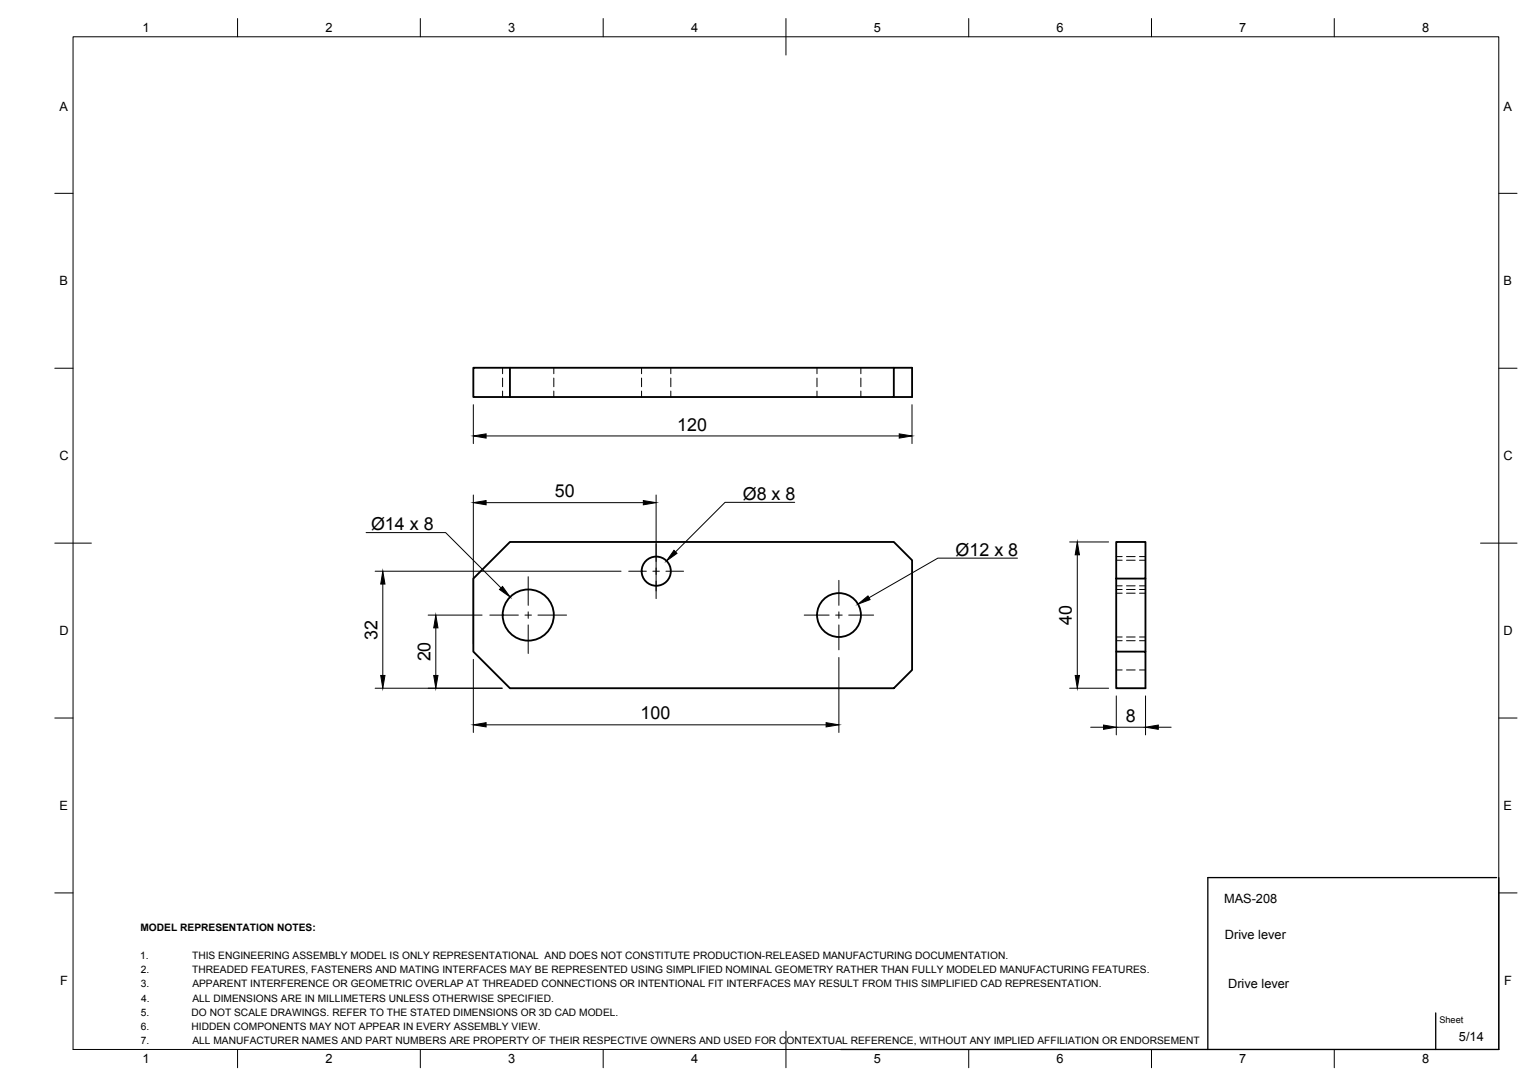
ISO-10303-21;
HEADER;
/* Generated by software containing ST-Developer
 * from STEP Tools, Inc. (www.steptools.com) 
 */

FILE_DESCRIPTION(
/* description */ ('Independent vertical20-tooth ratchet advance with repeated integral-c
ounterweight gravity pawls, swinging drive lever, bronze sleeves and f
ully retained axle stacks.18degpertooth. Native revolutes; geometric c
ycle checking rather than automatic contact/rolling dynamics. Gravity 
closing checked from actual pawl center of mass. Backplate/foot suppor
ts unit. Fits, torque, holding force, wear and life unassigned.'),
/* implementation_level */ '2;1');

FILE_NAME(
/* name */ 'Drive lever.step',
/* time_stamp */ '2026-11-09T06:25:53-08:00',
/* author */ (''),
/* organization */ (''),
/* preprocessor_version */ 'ST-DEVELOPER v20.2',
/* originating_system */ 'Autodesk Translation Framework v15.17.0.0',
/* authorisation */ '');

FILE_SCHEMA (('AUTOMOTIVE_DESIGN { 1 0 10303 214 3 1 1 }'));
ENDSEC;

DATA;
#10=MECHANICAL_DESIGN_GEOMETRIC_PRESENTATION_REPRESENTATION('',(#125),#4643);
#97=SHAPE_REPRESENTATION_RELATIONSHIP('SRR','None',#4702,#111);
#111=ADVANCED_BREP_SHAPE_REPRESENTATION('',(#139),#4631);
#125=STYLED_ITEM('',(#4781),#139);
#139=MANIFOLD_SOLID_BREP('Body1',#2661);
#165=FACE_BOUND('',#538,.T.);
#166=FACE_BOUND('',#539,.T.);
#167=FACE_BOUND('',#540,.T.);
#168=FACE_BOUND('',#542,.T.);
#169=FACE_BOUND('',#543,.T.);
#170=FACE_BOUND('',#544,.T.);
#244=PLANE('',#2914);
#245=PLANE('',#2915);
#246=PLANE('',#2916);
#247=PLANE('',#2917);
#248=PLANE('',#2918);
#249=PLANE('',#2919);
#250=PLANE('',#2920);
#251=PLANE('',#2921);
#252=PLANE('',#2922);
#253=PLANE('',#2923);
#363=FACE_OUTER_BOUND('',#526,.T.);
#364=FACE_OUTER_BOUND('',#527,.T.);
#365=FACE_OUTER_BOUND('',#528,.T.);
#366=FACE_OUTER_BOUND('',#529,.T.);
#367=FACE_OUTER_BOUND('',#530,.T.);
#368=FACE_OUTER_BOUND('',#531,.T.);
#369=FACE_OUTER_BOUND('',#532,.T.);
#370=FACE_OUTER_BOUND('',#533,.T.);
#371=FACE_OUTER_BOUND('',#534,.T.);
#372=FACE_OUTER_BOUND('',#535,.T.);
#373=FACE_OUTER_BOUND('',#536,.T.);
#374=FACE_OUTER_BOUND('',#537,.T.);
#375=FACE_OUTER_BOUND('',#541,.T.);
#526=EDGE_LOOP('',(#2131,#2132,#2133,#2134));
#527=EDGE_LOOP('',(#2135,#2136,#2137,#2138));
#528=EDGE_LOOP('',(#2139,#2140,#2141,#2142));
#529=EDGE_LOOP('',(#2143,#2144,#2145,#2146));
#530=EDGE_LOOP('',(#2147,#2148,#2149,#2150));
#531=EDGE_LOOP('',(#2151,#2152,#2153,#2154));
#532=EDGE_LOOP('',(#2155,#2156,#2157,#2158));
#533=EDGE_LOOP('',(#2159,#2160,#2161,#2162));
#534=EDGE_LOOP('',(#2163,#2164,#2165,#2166));
#535=EDGE_LOOP('',(#2167,#2168,#2169,#2170));
#536=EDGE_LOOP('',(#2171,#2172,#2173,#2174));
#537=EDGE_LOOP('',(#2175,#2176,#2177,#2178,#2179,#2180,#2181,#2182));
#538=EDGE_LOOP('',(#2183));
#539=EDGE_LOOP('',(#2184));
#540=EDGE_LOOP('',(#2185));
#541=EDGE_LOOP('',(#2186,#2187,#2188,#2189,#2190,#2191,#2192,#2193));
#542=EDGE_LOOP('',(#2194));
#543=EDGE_LOOP('',(#2195));
#544=EDGE_LOOP('',(#2196));
#794=LINE('',#4209,#1056);
#795=LINE('',#4215,#1057);
#796=LINE('',#4221,#1058);
#797=LINE('',#4226,#1059);
#798=LINE('',#4228,#1060);
#799=LINE('',#4230,#1061);
#800=LINE('',#4231,#1062);
#801=LINE('',#4234,#1063);
#802=LINE('',#4236,#1064);
#803=LINE('',#4237,#1065);
#804=LINE('',#4240,#1066);
#805=LINE('',#4242,#1067);
#806=LINE('',#4243,#1068);
#807=LINE('',#4246,#1069);
#808=LINE('',#4248,#1070);
#809=LINE('',#4249,#1071);
#810=LINE('',#4252,#1072);
#811=LINE('',#4254,#1073);
#812=LINE('',#4255,#1074);
#813=LINE('',#4258,#1075);
#814=LINE('',#4260,#1076);
#815=LINE('',#4261,#1077);
#816=LINE('',#4264,#1078);
#817=LINE('',#4266,#1079);
#818=LINE('',#4267,#1080);
#819=LINE('',#4269,#1081);
#820=LINE('',#4270,#1082);
#1056=VECTOR('',#3396,7.);
#1057=VECTOR('',#3403,4.);
#1058=VECTOR('',#3410,6.);
#1059=VECTOR('',#3415,10.);
#1060=VECTOR('',#3416,10.);
#1061=VECTOR('',#3417,10.);
#1062=VECTOR('',#3418,10.);
#1063=VECTOR('',#3421,10.);
#1064=VECTOR('',#3422,10.);
#1065=VECTOR('',#3423,10.);
#1066=VECTOR('',#3426,10.);
#1067=VECTOR('',#3427,10.);
#1068=VECTOR('',#3428,10.);
#1069=VECTOR('',#3431,10.);
#1070=VECTOR('',#3432,10.);
#1071=VECTOR('',#3433,10.);
#1072=VECTOR('',#3436,10.);
#1073=VECTOR('',#3437,10.);
#1074=VECTOR('',#3438,10.);
#1075=VECTOR('',#3441,10.);
#1076=VECTOR('',#3442,10.);
#1077=VECTOR('',#3443,10.);
#1078=VECTOR('',#3446,10.);
#1079=VECTOR('',#3447,10.);
#1080=VECTOR('',#3448,10.);
#1081=VECTOR('',#3451,10.);
#1082=VECTOR('',#3452,10.);
#1181=CIRCLE('',#2906,7.);
#1182=CIRCLE('',#2907,7.);
#1183=CIRCLE('',#2909,4.);
#1184=CIRCLE('',#2910,4.);
#1185=CIRCLE('',#2912,6.);
#1186=CIRCLE('',#2913,6.);
#1351=VERTEX_POINT('',#4206);
#1352=VERTEX_POINT('',#4208);
#1353=VERTEX_POINT('',#4212);
#1354=VERTEX_POINT('',#4214);
#1355=VERTEX_POINT('',#4218);
#1356=VERTEX_POINT('',#4220);
#1357=VERTEX_POINT('',#4224);
#1358=VERTEX_POINT('',#4225);
#1359=VERTEX_POINT('',#4227);
#1360=VERTEX_POINT('',#4229);
#1361=VERTEX_POINT('',#4233);
#1362=VERTEX_POINT('',#4235);
#1363=VERTEX_POINT('',#4239);
#1364=VERTEX_POINT('',#4241);
#1365=VERTEX_POINT('',#4245);
#1366=VERTEX_POINT('',#4247);
#1367=VERTEX_POINT('',#4251);
#1368=VERTEX_POINT('',#4253);
#1369=VERTEX_POINT('',#4257);
#1370=VERTEX_POINT('',#4259);
#1371=VERTEX_POINT('',#4263);
#1372=VERTEX_POINT('',#4265);
#1630=EDGE_CURVE('',#1351,#1351,#1181,.T.);
#1631=EDGE_CURVE('',#1351,#1352,#794,.T.);
#1632=EDGE_CURVE('',#1352,#1352,#1182,.T.);
#1633=EDGE_CURVE('',#1353,#1353,#1183,.T.);
#1634=EDGE_CURVE('',#1353,#1354,#795,.T.);
#1635=EDGE_CURVE('',#1354,#1354,#1184,.T.);
#1636=EDGE_CURVE('',#1355,#1355,#1185,.T.);
#1637=EDGE_CURVE('',#1355,#1356,#796,.T.);
#1638=EDGE_CURVE('',#1356,#1356,#1186,.T.);
#1639=EDGE_CURVE('',#1357,#1358,#797,.T.);
#1640=EDGE_CURVE('',#1358,#1359,#798,.T.);
#1641=EDGE_CURVE('',#1360,#1359,#799,.T.);
#1642=EDGE_CURVE('',#1357,#1360,#800,.T.);
#1643=EDGE_CURVE('',#1361,#1357,#801,.T.);
#1644=EDGE_CURVE('',#1362,#1360,#802,.T.);
#1645=EDGE_CURVE('',#1361,#1362,#803,.T.);
#1646=EDGE_CURVE('',#1363,#1361,#804,.T.);
#1647=EDGE_CURVE('',#1364,#1362,#805,.T.);
#1648=EDGE_CURVE('',#1363,#1364,#806,.T.);
#1649=EDGE_CURVE('',#1365,#1363,#807,.T.);
#1650=EDGE_CURVE('',#1366,#1364,#808,.T.);
#1651=EDGE_CURVE('',#1365,#1366,#809,.T.);
#1652=EDGE_CURVE('',#1367,#1365,#810,.T.);
#1653=EDGE_CURVE('',#1368,#1366,#811,.T.);
#1654=EDGE_CURVE('',#1367,#1368,#812,.T.);
#1655=EDGE_CURVE('',#1369,#1367,#813,.T.);
#1656=EDGE_CURVE('',#1370,#1368,#814,.T.);
#1657=EDGE_CURVE('',#1369,#1370,#815,.T.);
#1658=EDGE_CURVE('',#1371,#1369,#816,.T.);
#1659=EDGE_CURVE('',#1372,#1370,#817,.T.);
#1660=EDGE_CURVE('',#1371,#1372,#818,.T.);
#1661=EDGE_CURVE('',#1358,#1371,#819,.T.);
#1662=EDGE_CURVE('',#1359,#1372,#820,.T.);
#2131=ORIENTED_EDGE('',*,*,#1630,.F.);
#2132=ORIENTED_EDGE('',*,*,#1631,.T.);
#2133=ORIENTED_EDGE('',*,*,#1632,.F.);
#2134=ORIENTED_EDGE('',*,*,#1631,.F.);
#2135=ORIENTED_EDGE('',*,*,#1633,.F.);
#2136=ORIENTED_EDGE('',*,*,#1634,.T.);
#2137=ORIENTED_EDGE('',*,*,#1635,.F.);
#2138=ORIENTED_EDGE('',*,*,#1634,.F.);
#2139=ORIENTED_EDGE('',*,*,#1636,.F.);
#2140=ORIENTED_EDGE('',*,*,#1637,.T.);
#2141=ORIENTED_EDGE('',*,*,#1638,.F.);
#2142=ORIENTED_EDGE('',*,*,#1637,.F.);
#2143=ORIENTED_EDGE('',*,*,#1639,.T.);
#2144=ORIENTED_EDGE('',*,*,#1640,.T.);
#2145=ORIENTED_EDGE('',*,*,#1641,.F.);
#2146=ORIENTED_EDGE('',*,*,#1642,.F.);
#2147=ORIENTED_EDGE('',*,*,#1643,.T.);
#2148=ORIENTED_EDGE('',*,*,#1642,.T.);
#2149=ORIENTED_EDGE('',*,*,#1644,.F.);
#2150=ORIENTED_EDGE('',*,*,#1645,.F.);
#2151=ORIENTED_EDGE('',*,*,#1646,.T.);
#2152=ORIENTED_EDGE('',*,*,#1645,.T.);
#2153=ORIENTED_EDGE('',*,*,#1647,.F.);
#2154=ORIENTED_EDGE('',*,*,#1648,.F.);
#2155=ORIENTED_EDGE('',*,*,#1649,.T.);
#2156=ORIENTED_EDGE('',*,*,#1648,.T.);
#2157=ORIENTED_EDGE('',*,*,#1650,.F.);
#2158=ORIENTED_EDGE('',*,*,#1651,.F.);
#2159=ORIENTED_EDGE('',*,*,#1652,.T.);
#2160=ORIENTED_EDGE('',*,*,#1651,.T.);
#2161=ORIENTED_EDGE('',*,*,#1653,.F.);
#2162=ORIENTED_EDGE('',*,*,#1654,.F.);
#2163=ORIENTED_EDGE('',*,*,#1655,.T.);
#2164=ORIENTED_EDGE('',*,*,#1654,.T.);
#2165=ORIENTED_EDGE('',*,*,#1656,.F.);
#2166=ORIENTED_EDGE('',*,*,#1657,.F.);
#2167=ORIENTED_EDGE('',*,*,#1658,.T.);
#2168=ORIENTED_EDGE('',*,*,#1657,.T.);
#2169=ORIENTED_EDGE('',*,*,#1659,.F.);
#2170=ORIENTED_EDGE('',*,*,#1660,.F.);
#2171=ORIENTED_EDGE('',*,*,#1661,.T.);
#2172=ORIENTED_EDGE('',*,*,#1660,.T.);
#2173=ORIENTED_EDGE('',*,*,#1662,.F.);
#2174=ORIENTED_EDGE('',*,*,#1640,.F.);
#2175=ORIENTED_EDGE('',*,*,#1662,.T.);
#2176=ORIENTED_EDGE('',*,*,#1659,.T.);
#2177=ORIENTED_EDGE('',*,*,#1656,.T.);
#2178=ORIENTED_EDGE('',*,*,#1653,.T.);
#2179=ORIENTED_EDGE('',*,*,#1650,.T.);
#2180=ORIENTED_EDGE('',*,*,#1647,.T.);
#2181=ORIENTED_EDGE('',*,*,#1644,.T.);
#2182=ORIENTED_EDGE('',*,*,#1641,.T.);
#2183=ORIENTED_EDGE('',*,*,#1630,.T.);
#2184=ORIENTED_EDGE('',*,*,#1633,.T.);
#2185=ORIENTED_EDGE('',*,*,#1636,.T.);
#2186=ORIENTED_EDGE('',*,*,#1661,.F.);
#2187=ORIENTED_EDGE('',*,*,#1639,.F.);
#2188=ORIENTED_EDGE('',*,*,#1643,.F.);
#2189=ORIENTED_EDGE('',*,*,#1646,.F.);
#2190=ORIENTED_EDGE('',*,*,#1649,.F.);
#2191=ORIENTED_EDGE('',*,*,#1652,.F.);
#2192=ORIENTED_EDGE('',*,*,#1655,.F.);
#2193=ORIENTED_EDGE('',*,*,#1658,.F.);
#2194=ORIENTED_EDGE('',*,*,#1632,.T.);
#2195=ORIENTED_EDGE('',*,*,#1635,.T.);
#2196=ORIENTED_EDGE('',*,*,#1638,.T.);
#2480=CYLINDRICAL_SURFACE('',#2905,7.);
#2481=CYLINDRICAL_SURFACE('',#2908,4.);
#2482=CYLINDRICAL_SURFACE('',#2911,6.);
#2569=ADVANCED_FACE('',(#363),#2480,.F.);
#2570=ADVANCED_FACE('',(#364),#2481,.F.);
#2571=ADVANCED_FACE('',(#365),#2482,.F.);
#2572=ADVANCED_FACE('',(#366),#244,.T.);
#2573=ADVANCED_FACE('',(#367),#245,.T.);
#2574=ADVANCED_FACE('',(#368),#246,.T.);
#2575=ADVANCED_FACE('',(#369),#247,.T.);
#2576=ADVANCED_FACE('',(#370),#248,.T.);
#2577=ADVANCED_FACE('',(#371),#249,.T.);
#2578=ADVANCED_FACE('',(#372),#250,.T.);
#2579=ADVANCED_FACE('',(#373),#251,.T.);
#2580=ADVANCED_FACE('',(#374,#165,#166,#167),#252,.T.);
#2581=ADVANCED_FACE('',(#375,#168,#169,#170),#253,.F.);
#2661=CLOSED_SHELL('',(#2569,#2570,#2571,#2572,#2573,#2574,#2575,#2576,
#2577,#2578,#2579,#2580,#2581));
#2904=AXIS2_PLACEMENT_3D('',#4204,#3390,#3391);
#2905=AXIS2_PLACEMENT_3D('',#4205,#3392,#3393);
#2906=AXIS2_PLACEMENT_3D('',#4207,#3394,#3395);
#2907=AXIS2_PLACEMENT_3D('',#4210,#3397,#3398);
#2908=AXIS2_PLACEMENT_3D('',#4211,#3399,#3400);
#2909=AXIS2_PLACEMENT_3D('',#4213,#3401,#3402);
#2910=AXIS2_PLACEMENT_3D('',#4216,#3404,#3405);
#2911=AXIS2_PLACEMENT_3D('',#4217,#3406,#3407);
#2912=AXIS2_PLACEMENT_3D('',#4219,#3408,#3409);
#2913=AXIS2_PLACEMENT_3D('',#4222,#3411,#3412);
#2914=AXIS2_PLACEMENT_3D('',#4223,#3413,#3414);
#2915=AXIS2_PLACEMENT_3D('',#4232,#3419,#3420);
#2916=AXIS2_PLACEMENT_3D('',#4238,#3424,#3425);
#2917=AXIS2_PLACEMENT_3D('',#4244,#3429,#3430);
#2918=AXIS2_PLACEMENT_3D('',#4250,#3434,#3435);
#2919=AXIS2_PLACEMENT_3D('',#4256,#3439,#3440);
#2920=AXIS2_PLACEMENT_3D('',#4262,#3444,#3445);
#2921=AXIS2_PLACEMENT_3D('',#4268,#3449,#3450);
#2922=AXIS2_PLACEMENT_3D('',#4271,#3453,#3454);
#2923=AXIS2_PLACEMENT_3D('',#4272,#3455,#3456);
#3390=DIRECTION('axis',(0.,0.,1.));
#3391=DIRECTION('refdir',(1.,0.,0.));
#3392=DIRECTION('center_axis',(0.,0.,-1.));
#3393=DIRECTION('ref_axis',(1.,0.,0.));
#3394=DIRECTION('center_axis',(0.,0.,-1.));
#3395=DIRECTION('ref_axis',(1.,0.,0.));
#3396=DIRECTION('',(0.,0.,-1.));
#3397=DIRECTION('center_axis',(0.,0.,1.));
#3398=DIRECTION('ref_axis',(1.,0.,0.));
#3399=DIRECTION('center_axis',(0.,0.,-1.));
#3400=DIRECTION('ref_axis',(1.,0.,0.));
#3401=DIRECTION('center_axis',(0.,0.,-1.));
#3402=DIRECTION('ref_axis',(1.,0.,0.));
#3403=DIRECTION('',(0.,0.,-1.));
#3404=DIRECTION('center_axis',(0.,0.,1.));
#3405=DIRECTION('ref_axis',(1.,0.,0.));
#3406=DIRECTION('center_axis',(0.,0.,-1.));
#3407=DIRECTION('ref_axis',(1.,0.,0.));
#3408=DIRECTION('center_axis',(0.,0.,-1.));
#3409=DIRECTION('ref_axis',(1.,0.,0.));
#3410=DIRECTION('',(0.,0.,-1.));
#3411=DIRECTION('center_axis',(0.,0.,1.));
#3412=DIRECTION('ref_axis',(1.,0.,0.));
#3413=DIRECTION('center_axis',(-1.,0.,0.));
#3414=DIRECTION('ref_axis',(0.,-1.,0.));
#3415=DIRECTION('',(0.,-1.,0.));
#3416=DIRECTION('',(0.,0.,1.));
#3417=DIRECTION('',(0.,-1.,0.));
#3418=DIRECTION('',(0.,0.,1.));
#3419=DIRECTION('center_axis',(-0.707106781186548,0.707106781186548,0.));
#3420=DIRECTION('ref_axis',(-0.707106781186548,-0.707106781186548,0.));
#3421=DIRECTION('',(-0.707106781186547,-0.707106781186547,0.));
#3422=DIRECTION('',(-0.707106781186547,-0.707106781186547,0.));
#3423=DIRECTION('',(0.,0.,1.));
#3424=DIRECTION('center_axis',(0.,1.,0.));
#3425=DIRECTION('ref_axis',(-1.,0.,0.));
#3426=DIRECTION('',(-1.,0.,0.));
#3427=DIRECTION('',(-1.,0.,0.));
#3428=DIRECTION('',(0.,0.,1.));
#3429=DIRECTION('center_axis',(0.707106781186548,0.707106781186548,0.));
#3430=DIRECTION('ref_axis',(-0.707106781186548,0.707106781186548,0.));
#3431=DIRECTION('',(-0.707106781186547,0.707106781186547,0.));
#3432=DIRECTION('',(-0.707106781186547,0.707106781186547,0.));
#3433=DIRECTION('',(0.,0.,1.));
#3434=DIRECTION('center_axis',(1.,0.,0.));
#3435=DIRECTION('ref_axis',(0.,1.,0.));
#3436=DIRECTION('',(0.,1.,0.));
#3437=DIRECTION('',(0.,1.,0.));
#3438=DIRECTION('',(0.,0.,1.));
#3439=DIRECTION('center_axis',(0.707106781186548,-0.707106781186548,0.));
#3440=DIRECTION('ref_axis',(0.707106781186548,0.707106781186548,0.));
#3441=DIRECTION('',(0.707106781186547,0.707106781186547,0.));
#3442=DIRECTION('',(0.707106781186547,0.707106781186547,0.));
#3443=DIRECTION('',(0.,0.,1.));
#3444=DIRECTION('center_axis',(0.,-1.,0.));
#3445=DIRECTION('ref_axis',(1.,0.,0.));
#3446=DIRECTION('',(1.,0.,0.));
#3447=DIRECTION('',(1.,0.,0.));
#3448=DIRECTION('',(0.,0.,1.));
#3449=DIRECTION('center_axis',(-0.707106781186548,-0.707106781186548,0.));
#3450=DIRECTION('ref_axis',(0.707106781186548,-0.707106781186548,0.));
#3451=DIRECTION('',(0.707106781186547,-0.707106781186547,0.));
#3452=DIRECTION('',(0.707106781186547,-0.707106781186547,0.));
#3453=DIRECTION('center_axis',(0.,0.,1.));
#3454=DIRECTION('ref_axis',(1.,0.,0.));
#3455=DIRECTION('center_axis',(0.,0.,1.));
#3456=DIRECTION('ref_axis',(1.,0.,0.));
#4204=CARTESIAN_POINT('',(0.,0.,0.));
#4205=CARTESIAN_POINT('Origin',(85.,0.,4.));
#4206=CARTESIAN_POINT('',(78.,8.57252759403147E-16,8.));
#4207=CARTESIAN_POINT('Origin',(85.,0.,8.));
#4208=CARTESIAN_POINT('',(78.,8.57252759403147E-16,0.));
#4209=CARTESIAN_POINT('',(78.,8.57252759403147E-16,4.));
#4210=CARTESIAN_POINT('Origin',(85.,0.,0.));
#4211=CARTESIAN_POINT('Origin',(50.,12.,4.));
#4212=CARTESIAN_POINT('',(46.,12.,8.));
#4213=CARTESIAN_POINT('Origin',(50.,12.,8.));
#4214=CARTESIAN_POINT('',(46.,12.,0.));
#4215=CARTESIAN_POINT('',(46.,12.,4.));
#4216=CARTESIAN_POINT('Origin',(50.,12.,0.));
#4217=CARTESIAN_POINT('Origin',(0.,0.,4.));
#4218=CARTESIAN_POINT('',(-6.,7.34788079488412E-16,8.));
#4219=CARTESIAN_POINT('Origin',(0.,0.,8.));
#4220=CARTESIAN_POINT('',(-6.,7.34788079488412E-16,0.));
#4221=CARTESIAN_POINT('',(-6.,7.34788079488412E-16,4.));
#4222=CARTESIAN_POINT('Origin',(0.,0.,0.));
#4223=CARTESIAN_POINT('Origin',(-20.,15.,0.));
#4224=CARTESIAN_POINT('',(-20.,15.,0.));
#4225=CARTESIAN_POINT('',(-20.,-15.,0.));
#4226=CARTESIAN_POINT('',(-20.,15.,0.));
#4227=CARTESIAN_POINT('',(-20.,-15.,8.));
#4228=CARTESIAN_POINT('',(-20.,-15.,0.));
#4229=CARTESIAN_POINT('',(-20.,15.,8.));
#4230=CARTESIAN_POINT('',(-20.,15.,8.));
#4231=CARTESIAN_POINT('',(-20.,15.,0.));
#4232=CARTESIAN_POINT('Origin',(-15.,20.,0.));
#4233=CARTESIAN_POINT('',(-15.,20.,0.));
#4234=CARTESIAN_POINT('',(-15.,20.,0.));
#4235=CARTESIAN_POINT('',(-15.,20.,8.));
#4236=CARTESIAN_POINT('',(-15.,20.,8.));
#4237=CARTESIAN_POINT('',(-15.,20.,0.));
#4238=CARTESIAN_POINT('Origin',(90.,20.,0.));
#4239=CARTESIAN_POINT('',(90.,20.,0.));
#4240=CARTESIAN_POINT('',(90.,20.,0.));
#4241=CARTESIAN_POINT('',(90.,20.,8.));
#4242=CARTESIAN_POINT('',(90.,20.,8.));
#4243=CARTESIAN_POINT('',(90.,20.,0.));
#4244=CARTESIAN_POINT('Origin',(100.,10.,0.));
#4245=CARTESIAN_POINT('',(100.,10.,0.));
#4246=CARTESIAN_POINT('',(100.,10.,0.));
#4247=CARTESIAN_POINT('',(100.,10.,8.));
#4248=CARTESIAN_POINT('',(100.,10.,8.));
#4249=CARTESIAN_POINT('',(100.,10.,0.));
#4250=CARTESIAN_POINT('Origin',(100.,-10.,0.));
#4251=CARTESIAN_POINT('',(100.,-10.,0.));
#4252=CARTESIAN_POINT('',(100.,-10.,0.));
#4253=CARTESIAN_POINT('',(100.,-10.,8.));
#4254=CARTESIAN_POINT('',(100.,-10.,8.));
#4255=CARTESIAN_POINT('',(100.,-10.,0.));
#4256=CARTESIAN_POINT('Origin',(90.,-20.,0.));
#4257=CARTESIAN_POINT('',(90.,-20.,0.));
#4258=CARTESIAN_POINT('',(90.,-20.,0.));
#4259=CARTESIAN_POINT('',(90.,-20.,8.));
#4260=CARTESIAN_POINT('',(90.,-20.,8.));
#4261=CARTESIAN_POINT('',(90.,-20.,0.));
#4262=CARTESIAN_POINT('Origin',(-15.,-20.,0.));
#4263=CARTESIAN_POINT('',(-15.,-20.,0.));
#4264=CARTESIAN_POINT('',(-15.,-20.,0.));
#4265=CARTESIAN_POINT('',(-15.,-20.,8.));
#4266=CARTESIAN_POINT('',(-15.,-20.,8.));
#4267=CARTESIAN_POINT('',(-15.,-20.,0.));
#4268=CARTESIAN_POINT('Origin',(-20.,-15.,0.));
#4269=CARTESIAN_POINT('',(-20.,-15.,0.));
#4270=CARTESIAN_POINT('',(-20.,-15.,8.));
#4271=CARTESIAN_POINT('Origin',(40.,0.,8.));
#4272=CARTESIAN_POINT('Origin',(40.,0.,0.));
#4615=UNCERTAINTY_MEASURE_WITH_UNIT(LENGTH_MEASURE(0.01),#4644,
'DISTANCE_ACCURACY_VALUE',
'Maximum model space distance between geometric entities at asserted c
onnectivities');
#4627=UNCERTAINTY_MEASURE_WITH_UNIT(LENGTH_MEASURE(0.01),#4644,
'DISTANCE_ACCURACY_VALUE',
'Maximum model space distance between geometric entities at asserted c
onnectivities');
#4631=(
GEOMETRIC_REPRESENTATION_CONTEXT(3)
GLOBAL_UNCERTAINTY_ASSIGNED_CONTEXT((#4615))
GLOBAL_UNIT_ASSIGNED_CONTEXT((#4644,#4646,#4647))
REPRESENTATION_CONTEXT('','3D')
);
#4643=(
GEOMETRIC_REPRESENTATION_CONTEXT(3)
GLOBAL_UNCERTAINTY_ASSIGNED_CONTEXT((#4627))
GLOBAL_UNIT_ASSIGNED_CONTEXT((#4644,#4646,#4647))
REPRESENTATION_CONTEXT('','3D')
);
#4644=(
LENGTH_UNIT()
NAMED_UNIT(*)
SI_UNIT(.MILLI.,.METRE.)
);
#4646=(
NAMED_UNIT(*)
PLANE_ANGLE_UNIT()
SI_UNIT($,.RADIAN.)
);
#4647=(
NAMED_UNIT(*)
SI_UNIT($,.STERADIAN.)
SOLID_ANGLE_UNIT()
);
#4651=SHAPE_DEFINITION_REPRESENTATION(#4666,#4702);
#4666=PRODUCT_DEFINITION_SHAPE('',$,#4718);
#4702=SHAPE_REPRESENTATION('',(#2904),#4631);
#4714=PRODUCT_DEFINITION_CONTEXT('part definition',#4761,'design');
#4718=PRODUCT_DEFINITION('Drive lever','Drive lever',#4733,#4714);
#4733=PRODUCT_DEFINITION_FORMATION('',$,#4766);
#4761=APPLICATION_CONTEXT(
'Core Data for Automotive Mechanical Design Process');
#4762=PRODUCT_CONTEXT('part definition',#4761,'mechanical');
#4766=PRODUCT('Drive lever','Drive lever',$,(#4762));
#4781=PRESENTATION_STYLE_ASSIGNMENT((#4790));
#4790=SURFACE_STYLE_USAGE(.BOTH.,#4799);
#4799=SURFACE_SIDE_STYLE('',(#4808));
#4808=SURFACE_STYLE_FILL_AREA(#4817);
#4817=FILL_AREA_STYLE('Light blue',(#4826));
#4826=FILL_AREA_STYLE_COLOUR('Light blue',#4835);
#4835=COLOUR_RGB('Light blue',0.662745098039216,0.831372549019608,0.949019607843137);
ENDSEC;
END-ISO-10303-21;
